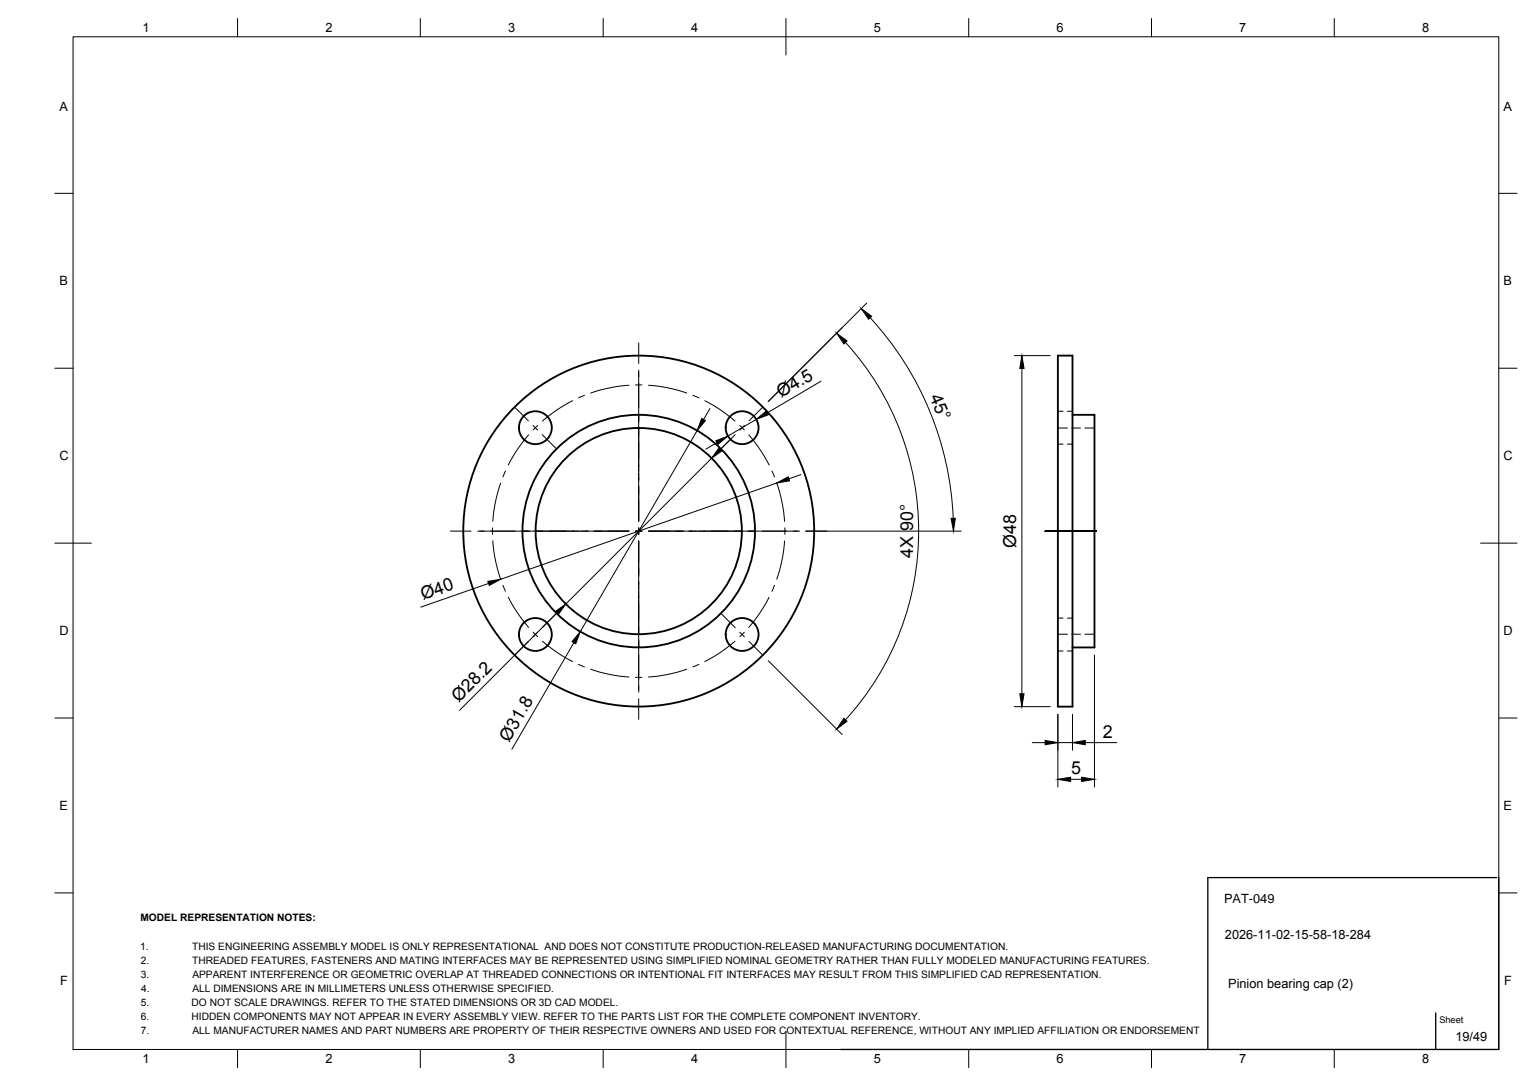
ISO-10303-21;
HEADER;
/* Generated by software containing ST-Developer
 * from STEP Tools, Inc. (www.steptools.com) 
 */

FILE_DESCRIPTION(
/* description */ ('Hand drill press frame (manual)'),
/* implementation_level */ '2;1');

FILE_NAME(
/* name */ 'Pinion bearing cap (2).step',
/* time_stamp */ '2026-10-28T03:25:28-07:00',
/* author */ (''),
/* organization */ (''),
/* preprocessor_version */ 'ST-DEVELOPER v20.2',
/* originating_system */ 'Autodesk Translation Framework v15.17.0.0',
/* authorisation */ '');

FILE_SCHEMA (('AUTOMOTIVE_DESIGN { 1 0 10303 214 3 1 1 }'));
ENDSEC;

DATA;
#10=MECHANICAL_DESIGN_GEOMETRIC_PRESENTATION_REPRESENTATION('',(#633),#33299);
#543=SHAPE_REPRESENTATION_RELATIONSHIP('SRR','None',#33502,#588);
#588=ADVANCED_BREP_SHAPE_REPRESENTATION('',(#685),#33264);
#633=STYLED_ITEM('',(#33814),#685);
#685=MANIFOLD_SOLID_BREP('Body1',#12651);
#814=FACE_BOUND('',#2321,.T.);
#815=FACE_BOUND('',#2325,.T.);
#816=FACE_BOUND('',#2326,.T.);
#817=FACE_BOUND('',#2327,.T.);
#818=FACE_BOUND('',#2328,.T.);
#819=FACE_BOUND('',#2329,.T.);
#820=FACE_BOUND('',#2331,.T.);
#821=FACE_BOUND('',#2332,.T.);
#822=FACE_BOUND('',#2333,.T.);
#823=FACE_BOUND('',#2334,.T.);
#824=FACE_BOUND('',#2335,.T.);
#1009=PLANE('',#13561);
#1010=PLANE('',#13568);
#1011=PLANE('',#13569);
#1532=FACE_OUTER_BOUND('',#2315,.T.);
#1533=FACE_OUTER_BOUND('',#2316,.T.);
#1534=FACE_OUTER_BOUND('',#2317,.T.);
#1535=FACE_OUTER_BOUND('',#2318,.T.);
#1536=FACE_OUTER_BOUND('',#2319,.T.);
#1537=FACE_OUTER_BOUND('',#2320,.T.);
#1538=FACE_OUTER_BOUND('',#2322,.T.);
#1539=FACE_OUTER_BOUND('',#2323,.T.);
#1540=FACE_OUTER_BOUND('',#2324,.T.);
#1541=FACE_OUTER_BOUND('',#2330,.T.);
#2315=EDGE_LOOP('',(#9353,#9354,#9355,#9356));
#2316=EDGE_LOOP('',(#9357,#9358,#9359,#9360));
#2317=EDGE_LOOP('',(#9361,#9362,#9363,#9364));
#2318=EDGE_LOOP('',(#9365,#9366,#9367,#9368));
#2319=EDGE_LOOP('',(#9369,#9370,#9371,#9372));
#2320=EDGE_LOOP('',(#9373));
#2321=EDGE_LOOP('',(#9374));
#2322=EDGE_LOOP('',(#9375,#9376,#9377,#9378));
#2323=EDGE_LOOP('',(#9379,#9380,#9381,#9382));
#2324=EDGE_LOOP('',(#9383));
#2325=EDGE_LOOP('',(#9384));
#2326=EDGE_LOOP('',(#9385));
#2327=EDGE_LOOP('',(#9386));
#2328=EDGE_LOOP('',(#9387));
#2329=EDGE_LOOP('',(#9388));
#2330=EDGE_LOOP('',(#9389));
#2331=EDGE_LOOP('',(#9390));
#2332=EDGE_LOOP('',(#9391));
#2333=EDGE_LOOP('',(#9392));
#2334=EDGE_LOOP('',(#9393));
#2335=EDGE_LOOP('',(#9394));
#3187=LINE('',#19064,#4352);
#3188=LINE('',#19070,#4353);
#3189=LINE('',#19076,#4354);
#3190=LINE('',#19082,#4355);
#3191=LINE('',#19088,#4356);
#3192=LINE('',#19095,#4357);
#3193=LINE('',#19101,#4358);
#4352=VECTOR('',#15390,0.225);
#4353=VECTOR('',#15397,0.225);
#4354=VECTOR('',#15404,0.225);
#4355=VECTOR('',#15411,0.225);
#4356=VECTOR('',#15418,1.59);
#4357=VECTOR('',#15427,1.41);
#4358=VECTOR('',#15434,2.4);
#5362=CIRCLE('',#13547,0.225);
#5363=CIRCLE('',#13548,0.225);
#5364=CIRCLE('',#13550,0.225);
#5365=CIRCLE('',#13551,0.225);
#5366=CIRCLE('',#13553,0.225);
#5367=CIRCLE('',#13554,0.225);
#5368=CIRCLE('',#13556,0.225);
#5369=CIRCLE('',#13557,0.225);
#5370=CIRCLE('',#13559,1.59);
#5371=CIRCLE('',#13560,1.59);
#5372=CIRCLE('',#13562,1.41);
#5373=CIRCLE('',#13564,1.41);
#5374=CIRCLE('',#13566,2.4);
#5375=CIRCLE('',#13567,2.4);
#5924=VERTEX_POINT('',#19061);
#5925=VERTEX_POINT('',#19063);
#5926=VERTEX_POINT('',#19067);
#5927=VERTEX_POINT('',#19069);
#5928=VERTEX_POINT('',#19073);
#5929=VERTEX_POINT('',#19075);
#5930=VERTEX_POINT('',#19079);
#5931=VERTEX_POINT('',#19081);
#5932=VERTEX_POINT('',#19085);
#5933=VERTEX_POINT('',#19087);
#5934=VERTEX_POINT('',#19091);
#5935=VERTEX_POINT('',#19094);
#5936=VERTEX_POINT('',#19098);
#5937=VERTEX_POINT('',#19100);
#7205=EDGE_CURVE('',#5924,#5924,#5362,.T.);
#7206=EDGE_CURVE('',#5924,#5925,#3187,.T.);
#7207=EDGE_CURVE('',#5925,#5925,#5363,.T.);
#7208=EDGE_CURVE('',#5926,#5926,#5364,.T.);
#7209=EDGE_CURVE('',#5926,#5927,#3188,.T.);
#7210=EDGE_CURVE('',#5927,#5927,#5365,.T.);
#7211=EDGE_CURVE('',#5928,#5928,#5366,.T.);
#7212=EDGE_CURVE('',#5928,#5929,#3189,.T.);
#7213=EDGE_CURVE('',#5929,#5929,#5367,.T.);
#7214=EDGE_CURVE('',#5930,#5930,#5368,.T.);
#7215=EDGE_CURVE('',#5930,#5931,#3190,.T.);
#7216=EDGE_CURVE('',#5931,#5931,#5369,.T.);
#7217=EDGE_CURVE('',#5932,#5932,#5370,.T.);
#7218=EDGE_CURVE('',#5932,#5933,#3191,.T.);
#7219=EDGE_CURVE('',#5933,#5933,#5371,.T.);
#7220=EDGE_CURVE('',#5934,#5934,#5372,.T.);
#7221=EDGE_CURVE('',#5934,#5935,#3192,.T.);
#7222=EDGE_CURVE('',#5935,#5935,#5373,.T.);
#7223=EDGE_CURVE('',#5936,#5936,#5374,.T.);
#7224=EDGE_CURVE('',#5936,#5937,#3193,.T.);
#7225=EDGE_CURVE('',#5937,#5937,#5375,.T.);
#9353=ORIENTED_EDGE('',*,*,#7205,.F.);
#9354=ORIENTED_EDGE('',*,*,#7206,.T.);
#9355=ORIENTED_EDGE('',*,*,#7207,.F.);
#9356=ORIENTED_EDGE('',*,*,#7206,.F.);
#9357=ORIENTED_EDGE('',*,*,#7208,.F.);
#9358=ORIENTED_EDGE('',*,*,#7209,.T.);
#9359=ORIENTED_EDGE('',*,*,#7210,.F.);
#9360=ORIENTED_EDGE('',*,*,#7209,.F.);
#9361=ORIENTED_EDGE('',*,*,#7211,.F.);
#9362=ORIENTED_EDGE('',*,*,#7212,.T.);
#9363=ORIENTED_EDGE('',*,*,#7213,.F.);
#9364=ORIENTED_EDGE('',*,*,#7212,.F.);
#9365=ORIENTED_EDGE('',*,*,#7214,.F.);
#9366=ORIENTED_EDGE('',*,*,#7215,.T.);
#9367=ORIENTED_EDGE('',*,*,#7216,.F.);
#9368=ORIENTED_EDGE('',*,*,#7215,.F.);
#9369=ORIENTED_EDGE('',*,*,#7217,.F.);
#9370=ORIENTED_EDGE('',*,*,#7218,.T.);
#9371=ORIENTED_EDGE('',*,*,#7219,.F.);
#9372=ORIENTED_EDGE('',*,*,#7218,.F.);
#9373=ORIENTED_EDGE('',*,*,#7217,.T.);
#9374=ORIENTED_EDGE('',*,*,#7220,.T.);
#9375=ORIENTED_EDGE('',*,*,#7220,.F.);
#9376=ORIENTED_EDGE('',*,*,#7221,.T.);
#9377=ORIENTED_EDGE('',*,*,#7222,.T.);
#9378=ORIENTED_EDGE('',*,*,#7221,.F.);
#9379=ORIENTED_EDGE('',*,*,#7223,.F.);
#9380=ORIENTED_EDGE('',*,*,#7224,.T.);
#9381=ORIENTED_EDGE('',*,*,#7225,.T.);
#9382=ORIENTED_EDGE('',*,*,#7224,.F.);
#9383=ORIENTED_EDGE('',*,*,#7223,.T.);
#9384=ORIENTED_EDGE('',*,*,#7219,.T.);
#9385=ORIENTED_EDGE('',*,*,#7216,.T.);
#9386=ORIENTED_EDGE('',*,*,#7213,.T.);
#9387=ORIENTED_EDGE('',*,*,#7210,.T.);
#9388=ORIENTED_EDGE('',*,*,#7207,.T.);
#9389=ORIENTED_EDGE('',*,*,#7225,.F.);
#9390=ORIENTED_EDGE('',*,*,#7222,.F.);
#9391=ORIENTED_EDGE('',*,*,#7214,.T.);
#9392=ORIENTED_EDGE('',*,*,#7211,.T.);
#9393=ORIENTED_EDGE('',*,*,#7208,.T.);
#9394=ORIENTED_EDGE('',*,*,#7205,.T.);
#11856=CYLINDRICAL_SURFACE('',#13546,0.225);
#11857=CYLINDRICAL_SURFACE('',#13549,0.225);
#11858=CYLINDRICAL_SURFACE('',#13552,0.225);
#11859=CYLINDRICAL_SURFACE('',#13555,0.225);
#11860=CYLINDRICAL_SURFACE('',#13558,1.59);
#11861=CYLINDRICAL_SURFACE('',#13563,1.41);
#11862=CYLINDRICAL_SURFACE('',#13565,2.4);
#12141=ADVANCED_FACE('',(#1532),#11856,.F.);
#12142=ADVANCED_FACE('',(#1533),#11857,.F.);
#12143=ADVANCED_FACE('',(#1534),#11858,.F.);
#12144=ADVANCED_FACE('',(#1535),#11859,.F.);
#12145=ADVANCED_FACE('',(#1536),#11860,.T.);
#12146=ADVANCED_FACE('',(#1537,#814),#1009,.T.);
#12147=ADVANCED_FACE('',(#1538),#11861,.F.);
#12148=ADVANCED_FACE('',(#1539),#11862,.T.);
#12149=ADVANCED_FACE('',(#1540,#815,#816,#817,#818,#819),#1010,.T.);
#12150=ADVANCED_FACE('',(#1541,#820,#821,#822,#823,#824),#1011,.F.);
#12651=CLOSED_SHELL('',(#12141,#12142,#12143,#12144,#12145,#12146,#12147,
#12148,#12149,#12150));
#13545=AXIS2_PLACEMENT_3D('',#19059,#15384,#15385);
#13546=AXIS2_PLACEMENT_3D('',#19060,#15386,#15387);
#13547=AXIS2_PLACEMENT_3D('',#19062,#15388,#15389);
#13548=AXIS2_PLACEMENT_3D('',#19065,#15391,#15392);
#13549=AXIS2_PLACEMENT_3D('',#19066,#15393,#15394);
#13550=AXIS2_PLACEMENT_3D('',#19068,#15395,#15396);
#13551=AXIS2_PLACEMENT_3D('',#19071,#15398,#15399);
#13552=AXIS2_PLACEMENT_3D('',#19072,#15400,#15401);
#13553=AXIS2_PLACEMENT_3D('',#19074,#15402,#15403);
#13554=AXIS2_PLACEMENT_3D('',#19077,#15405,#15406);
#13555=AXIS2_PLACEMENT_3D('',#19078,#15407,#15408);
#13556=AXIS2_PLACEMENT_3D('',#19080,#15409,#15410);
#13557=AXIS2_PLACEMENT_3D('',#19083,#15412,#15413);
#13558=AXIS2_PLACEMENT_3D('',#19084,#15414,#15415);
#13559=AXIS2_PLACEMENT_3D('',#19086,#15416,#15417);
#13560=AXIS2_PLACEMENT_3D('',#19089,#15419,#15420);
#13561=AXIS2_PLACEMENT_3D('',#19090,#15421,#15422);
#13562=AXIS2_PLACEMENT_3D('',#19092,#15423,#15424);
#13563=AXIS2_PLACEMENT_3D('',#19093,#15425,#15426);
#13564=AXIS2_PLACEMENT_3D('',#19096,#15428,#15429);
#13565=AXIS2_PLACEMENT_3D('',#19097,#15430,#15431);
#13566=AXIS2_PLACEMENT_3D('',#19099,#15432,#15433);
#13567=AXIS2_PLACEMENT_3D('',#19102,#15435,#15436);
#13568=AXIS2_PLACEMENT_3D('',#19103,#15437,#15438);
#13569=AXIS2_PLACEMENT_3D('',#19104,#15439,#15440);
#15384=DIRECTION('axis',(0.,0.,1.));
#15385=DIRECTION('refdir',(1.,0.,0.));
#15386=DIRECTION('center_axis',(0.,1.,0.));
#15387=DIRECTION('ref_axis',(1.,0.,0.));
#15388=DIRECTION('center_axis',(0.,1.,0.));
#15389=DIRECTION('ref_axis',(1.,0.,0.));
#15390=DIRECTION('',(0.,1.,0.));
#15391=DIRECTION('center_axis',(0.,-1.,0.));
#15392=DIRECTION('ref_axis',(1.,0.,0.));
#15393=DIRECTION('center_axis',(0.,1.,0.));
#15394=DIRECTION('ref_axis',(1.,0.,0.));
#15395=DIRECTION('center_axis',(0.,1.,0.));
#15396=DIRECTION('ref_axis',(1.,0.,0.));
#15397=DIRECTION('',(0.,1.,0.));
#15398=DIRECTION('center_axis',(0.,-1.,0.));
#15399=DIRECTION('ref_axis',(1.,0.,0.));
#15400=DIRECTION('center_axis',(0.,1.,0.));
#15401=DIRECTION('ref_axis',(1.,0.,0.));
#15402=DIRECTION('center_axis',(0.,1.,0.));
#15403=DIRECTION('ref_axis',(1.,0.,0.));
#15404=DIRECTION('',(0.,1.,0.));
#15405=DIRECTION('center_axis',(0.,-1.,0.));
#15406=DIRECTION('ref_axis',(1.,0.,0.));
#15407=DIRECTION('center_axis',(0.,1.,0.));
#15408=DIRECTION('ref_axis',(1.,0.,0.));
#15409=DIRECTION('center_axis',(0.,1.,0.));
#15410=DIRECTION('ref_axis',(1.,0.,0.));
#15411=DIRECTION('',(0.,1.,0.));
#15412=DIRECTION('center_axis',(0.,-1.,0.));
#15413=DIRECTION('ref_axis',(1.,0.,0.));
#15414=DIRECTION('center_axis',(0.,1.,0.));
#15415=DIRECTION('ref_axis',(1.,0.,0.));
#15416=DIRECTION('center_axis',(0.,1.,0.));
#15417=DIRECTION('ref_axis',(1.,0.,0.));
#15418=DIRECTION('',(0.,-1.,0.));
#15419=DIRECTION('center_axis',(0.,-1.,0.));
#15420=DIRECTION('ref_axis',(1.,0.,0.));
#15421=DIRECTION('center_axis',(0.,1.,0.));
#15422=DIRECTION('ref_axis',(1.,0.,0.));
#15423=DIRECTION('center_axis',(0.,-1.,0.));
#15424=DIRECTION('ref_axis',(1.,0.,0.));
#15425=DIRECTION('center_axis',(0.,1.,0.));
#15426=DIRECTION('ref_axis',(1.,0.,0.));
#15427=DIRECTION('',(0.,-1.,0.));
#15428=DIRECTION('center_axis',(0.,-1.,0.));
#15429=DIRECTION('ref_axis',(1.,0.,0.));
#15430=DIRECTION('center_axis',(0.,1.,0.));
#15431=DIRECTION('ref_axis',(1.,0.,0.));
#15432=DIRECTION('center_axis',(0.,1.,0.));
#15433=DIRECTION('ref_axis',(1.,0.,0.));
#15434=DIRECTION('',(0.,-1.,0.));
#15435=DIRECTION('center_axis',(0.,1.,0.));
#15436=DIRECTION('ref_axis',(1.,0.,0.));
#15437=DIRECTION('center_axis',(0.,1.,0.));
#15438=DIRECTION('ref_axis',(1.,0.,0.));
#15439=DIRECTION('center_axis',(0.,1.,0.));
#15440=DIRECTION('ref_axis',(1.,0.,0.));
#19059=CARTESIAN_POINT('',(0.,0.,0.));
#19060=CARTESIAN_POINT('Origin',(-4.66421356237309,1.9,18.5857864376269));
#19061=CARTESIAN_POINT('',(-4.88921356237309,2.,18.5857864376269));
#19062=CARTESIAN_POINT('Origin',(-4.66421356237309,2.,18.5857864376269));
#19063=CARTESIAN_POINT('',(-4.88921356237309,2.2,18.5857864376269));
#19064=CARTESIAN_POINT('',(-4.88921356237309,1.9,18.5857864376269));
#19065=CARTESIAN_POINT('Origin',(-4.66421356237309,2.2,18.5857864376269));
#19066=CARTESIAN_POINT('Origin',(-4.66421356237309,1.9,21.4142135623731));
#19067=CARTESIAN_POINT('',(-4.88921356237309,2.,21.4142135623731));
#19068=CARTESIAN_POINT('Origin',(-4.66421356237309,2.,21.4142135623731));
#19069=CARTESIAN_POINT('',(-4.88921356237309,2.2,21.4142135623731));
#19070=CARTESIAN_POINT('',(-4.88921356237309,1.9,21.4142135623731));
#19071=CARTESIAN_POINT('Origin',(-4.66421356237309,2.2,21.4142135623731));
#19072=CARTESIAN_POINT('Origin',(-1.8357864376269,1.9,21.4142135623731));
#19073=CARTESIAN_POINT('',(-2.0607864376269,2.,21.4142135623731));
#19074=CARTESIAN_POINT('Origin',(-1.8357864376269,2.,21.4142135623731));
#19075=CARTESIAN_POINT('',(-2.0607864376269,2.2,21.4142135623731));
#19076=CARTESIAN_POINT('',(-2.0607864376269,1.9,21.4142135623731));
#19077=CARTESIAN_POINT('Origin',(-1.8357864376269,2.2,21.4142135623731));
#19078=CARTESIAN_POINT('Origin',(-1.83578643762691,1.9,18.5857864376269));
#19079=CARTESIAN_POINT('',(-2.06078643762691,2.,18.5857864376269));
#19080=CARTESIAN_POINT('Origin',(-1.83578643762691,2.,18.5857864376269));
#19081=CARTESIAN_POINT('',(-2.06078643762691,2.2,18.5857864376269));
#19082=CARTESIAN_POINT('',(-2.06078643762691,1.9,18.5857864376269));
#19083=CARTESIAN_POINT('Origin',(-1.83578643762691,2.2,18.5857864376269));
#19084=CARTESIAN_POINT('Origin',(-3.25,2.2,20.));
#19085=CARTESIAN_POINT('',(-4.84,2.5,20.));
#19086=CARTESIAN_POINT('Origin',(-3.25,2.5,20.));
#19087=CARTESIAN_POINT('',(-4.84,2.2,20.));
#19088=CARTESIAN_POINT('',(-4.84,2.2,20.));
#19089=CARTESIAN_POINT('Origin',(-3.25,2.2,20.));
#19090=CARTESIAN_POINT('Origin',(-3.25,2.5,20.));
#19091=CARTESIAN_POINT('',(-4.66,2.5,20.));
#19092=CARTESIAN_POINT('Origin',(-3.25,2.5,20.));
#19093=CARTESIAN_POINT('Origin',(-3.25,2.,20.));
#19094=CARTESIAN_POINT('',(-4.66,2.,20.));
#19095=CARTESIAN_POINT('',(-4.66,2.,20.));
#19096=CARTESIAN_POINT('Origin',(-3.25,2.,20.));
#19097=CARTESIAN_POINT('Origin',(-3.25,2.,20.));
#19098=CARTESIAN_POINT('',(-5.65,2.2,20.));
#19099=CARTESIAN_POINT('Origin',(-3.25,2.2,20.));
#19100=CARTESIAN_POINT('',(-5.65,2.,20.));
#19101=CARTESIAN_POINT('',(-5.65,2.,20.));
#19102=CARTESIAN_POINT('Origin',(-3.25,2.,20.));
#19103=CARTESIAN_POINT('Origin',(-3.25,2.2,20.));
#19104=CARTESIAN_POINT('Origin',(-3.25,2.,20.));
#33212=UNCERTAINTY_MEASURE_WITH_UNIT(LENGTH_MEASURE(0.001),#33300,
'DISTANCE_ACCURACY_VALUE',
'Maximum model space distance between geometric entities at asserted c
onnectivities');
#33247=UNCERTAINTY_MEASURE_WITH_UNIT(LENGTH_MEASURE(0.001),#33300,
'DISTANCE_ACCURACY_VALUE',
'Maximum model space distance between geometric entities at asserted c
onnectivities');
#33264=(
GEOMETRIC_REPRESENTATION_CONTEXT(3)
GLOBAL_UNCERTAINTY_ASSIGNED_CONTEXT((#33212))
GLOBAL_UNIT_ASSIGNED_CONTEXT((#33300,#33302,#33303))
REPRESENTATION_CONTEXT('','3D')
);
#33299=(
GEOMETRIC_REPRESENTATION_CONTEXT(3)
GLOBAL_UNCERTAINTY_ASSIGNED_CONTEXT((#33247))
GLOBAL_UNIT_ASSIGNED_CONTEXT((#33300,#33302,#33303))
REPRESENTATION_CONTEXT('','3D')
);
#33300=(
LENGTH_UNIT()
NAMED_UNIT(*)
SI_UNIT(.CENTI.,.METRE.)
);
#33302=(
NAMED_UNIT(*)
PLANE_ANGLE_UNIT()
SI_UNIT($,.RADIAN.)
);
#33303=(
NAMED_UNIT(*)
SI_UNIT($,.STERADIAN.)
SOLID_ANGLE_UNIT()
);
#33320=SHAPE_DEFINITION_REPRESENTATION(#33371,#33502);
#33371=PRODUCT_DEFINITION_SHAPE('',$,#33554);
#33502=SHAPE_REPRESENTATION('',(#13545),#33264);
#33537=PRODUCT_DEFINITION_CONTEXT('part definition',#33692,'design');
#33554=PRODUCT_DEFINITION('Pinion bearing cap (2)',
'Pinion bearing cap (2)',#33605,#33537);
#33605=PRODUCT_DEFINITION_FORMATION('',$,#33710);
#33692=APPLICATION_CONTEXT(
'Core Data for Automotive Mechanical Design Process');
#33693=PRODUCT_CONTEXT('part definition',#33692,'mechanical');
#33710=PRODUCT('Pinion bearing cap (2)','Pinion bearing cap (2)',
'Pinion bearing cap (2)',(#33693));
#33808=COLOUR_RGB('Grey',0.48,0.52,0.57);
#33809=FILL_AREA_STYLE_COLOUR('',#33808);
#33810=FILL_AREA_STYLE('',(#33809));
#33811=SURFACE_STYLE_FILL_AREA(#33810);
#33812=SURFACE_SIDE_STYLE('',(#33811));
#33813=SURFACE_STYLE_USAGE(.BOTH.,#33812);
#33814=PRESENTATION_STYLE_ASSIGNMENT((#33813));
ENDSEC;
END-ISO-10303-21;
